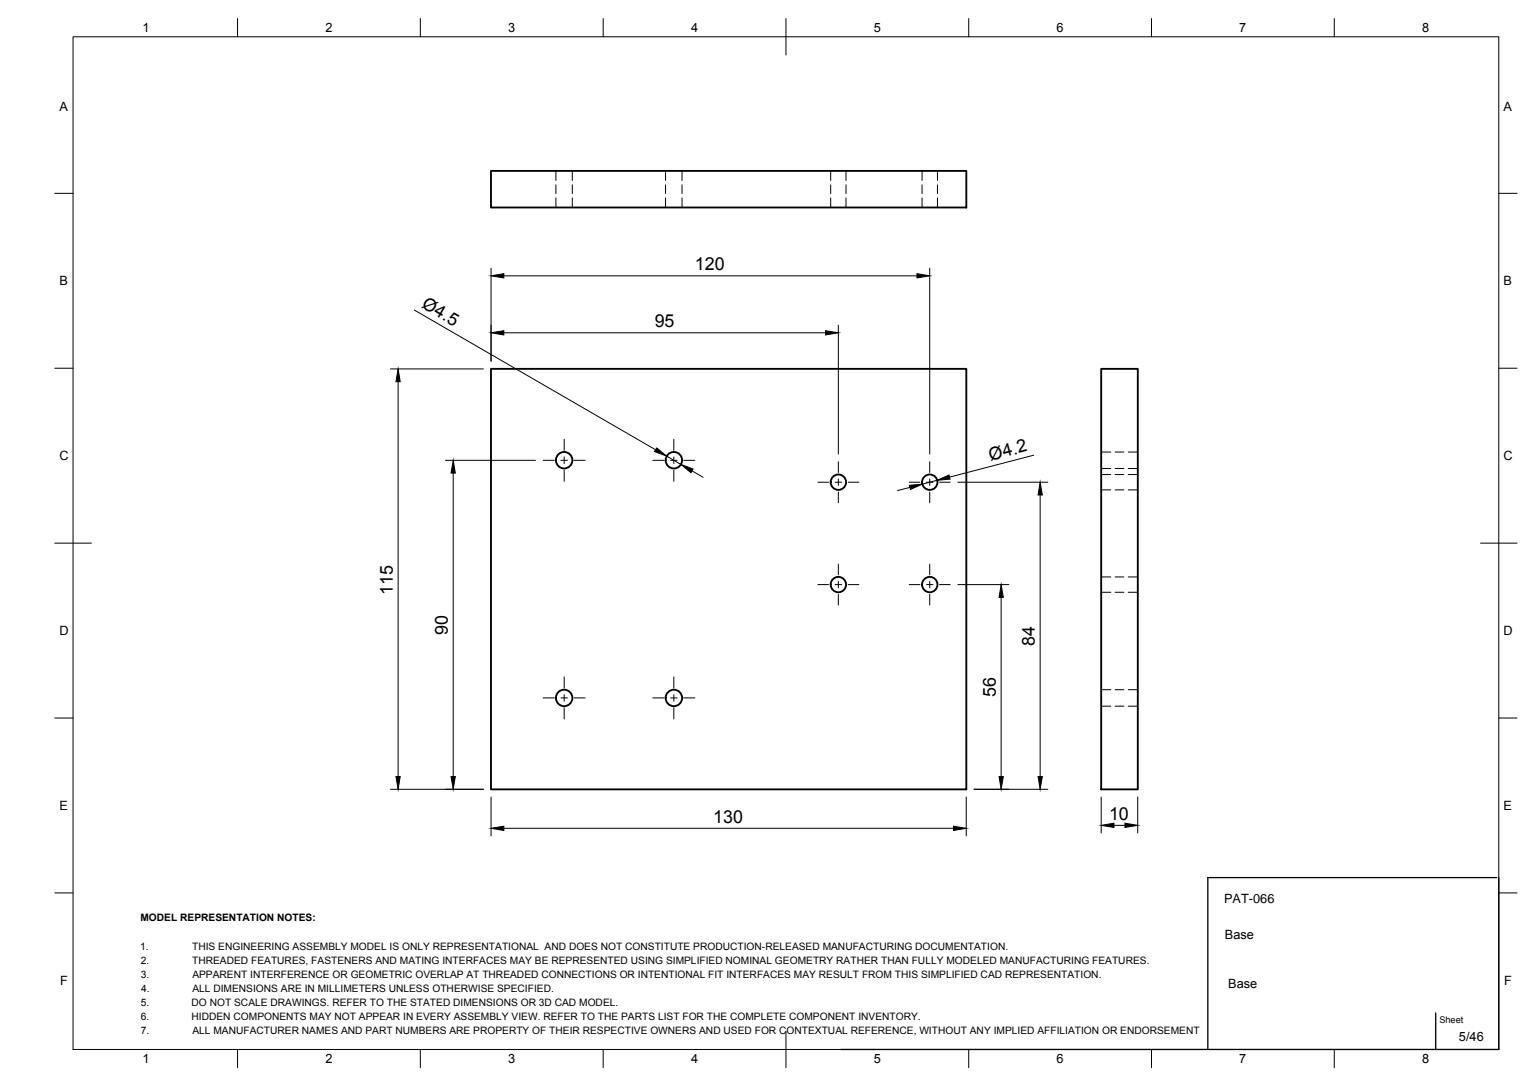
ISO-10303-21;
HEADER;
/* Generated by software containing ST-Developer
 * from STEP Tools, Inc. (www.steptools.com) 
 */

FILE_DESCRIPTION(
/* description */ ('Lever-operated bar clamp (toggle)'),
/* implementation_level */ '2;1');

FILE_NAME(
/* name */ 'Base.step',
/* time_stamp */ '2026-10-28T03:25:02-07:00',
/* author */ (''),
/* organization */ (''),
/* preprocessor_version */ 'ST-DEVELOPER v20.2',
/* originating_system */ 'Autodesk Translation Framework v15.17.0.0',
/* authorisation */ '');

FILE_SCHEMA (('AUTOMOTIVE_DESIGN { 1 0 10303 214 3 1 1 }'));
ENDSEC;

DATA;
#10=MECHANICAL_DESIGN_GEOMETRIC_PRESENTATION_REPRESENTATION('',(#410),#12413);
#334=SHAPE_REPRESENTATION_RELATIONSHIP('SRR','None',#12573,#372);
#372=ADVANCED_BREP_SHAPE_REPRESENTATION('',(#457),#12370);
#410=STYLED_ITEM('',(#12848),#457);
#457=MANIFOLD_SOLID_BREP('Body1',#6569);
#500=FACE_BOUND('',#1307,.T.);
#501=FACE_BOUND('',#1308,.T.);
#502=FACE_BOUND('',#1309,.T.);
#503=FACE_BOUND('',#1310,.T.);
#504=FACE_BOUND('',#1311,.T.);
#505=FACE_BOUND('',#1312,.T.);
#506=FACE_BOUND('',#1313,.T.);
#507=FACE_BOUND('',#1314,.T.);
#508=FACE_BOUND('',#1316,.T.);
#509=FACE_BOUND('',#1317,.T.);
#510=FACE_BOUND('',#1318,.T.);
#511=FACE_BOUND('',#1319,.T.);
#512=FACE_BOUND('',#1320,.T.);
#513=FACE_BOUND('',#1321,.T.);
#514=FACE_BOUND('',#1322,.T.);
#515=FACE_BOUND('',#1323,.T.);
#651=PLANE('',#7066);
#652=PLANE('',#7067);
#653=PLANE('',#7068);
#654=PLANE('',#7069);
#655=PLANE('',#7070);
#656=PLANE('',#7071);
#888=FACE_OUTER_BOUND('',#1294,.T.);
#889=FACE_OUTER_BOUND('',#1295,.T.);
#890=FACE_OUTER_BOUND('',#1296,.T.);
#891=FACE_OUTER_BOUND('',#1297,.T.);
#892=FACE_OUTER_BOUND('',#1298,.T.);
#893=FACE_OUTER_BOUND('',#1299,.T.);
#894=FACE_OUTER_BOUND('',#1300,.T.);
#895=FACE_OUTER_BOUND('',#1301,.T.);
#896=FACE_OUTER_BOUND('',#1302,.T.);
#897=FACE_OUTER_BOUND('',#1303,.T.);
#898=FACE_OUTER_BOUND('',#1304,.T.);
#899=FACE_OUTER_BOUND('',#1305,.T.);
#900=FACE_OUTER_BOUND('',#1306,.T.);
#901=FACE_OUTER_BOUND('',#1315,.T.);
#1294=EDGE_LOOP('',(#4421,#4422,#4423,#4424));
#1295=EDGE_LOOP('',(#4425,#4426,#4427,#4428));
#1296=EDGE_LOOP('',(#4429,#4430,#4431,#4432));
#1297=EDGE_LOOP('',(#4433,#4434,#4435,#4436));
#1298=EDGE_LOOP('',(#4437,#4438,#4439,#4440));
#1299=EDGE_LOOP('',(#4441,#4442,#4443,#4444));
#1300=EDGE_LOOP('',(#4445,#4446,#4447,#4448));
#1301=EDGE_LOOP('',(#4449,#4450,#4451,#4452));
#1302=EDGE_LOOP('',(#4453,#4454,#4455,#4456));
#1303=EDGE_LOOP('',(#4457,#4458,#4459,#4460));
#1304=EDGE_LOOP('',(#4461,#4462,#4463,#4464));
#1305=EDGE_LOOP('',(#4465,#4466,#4467,#4468));
#1306=EDGE_LOOP('',(#4469,#4470,#4471,#4472));
#1307=EDGE_LOOP('',(#4473));
#1308=EDGE_LOOP('',(#4474));
#1309=EDGE_LOOP('',(#4475));
#1310=EDGE_LOOP('',(#4476));
#1311=EDGE_LOOP('',(#4477));
#1312=EDGE_LOOP('',(#4478));
#1313=EDGE_LOOP('',(#4479));
#1314=EDGE_LOOP('',(#4480));
#1315=EDGE_LOOP('',(#4481,#4482,#4483,#4484));
#1316=EDGE_LOOP('',(#4485));
#1317=EDGE_LOOP('',(#4486));
#1318=EDGE_LOOP('',(#4487));
#1319=EDGE_LOOP('',(#4488));
#1320=EDGE_LOOP('',(#4489));
#1321=EDGE_LOOP('',(#4490));
#1322=EDGE_LOOP('',(#4491));
#1323=EDGE_LOOP('',(#4492));
#1851=LINE('',#10052,#2292);
#1852=LINE('',#10058,#2293);
#1853=LINE('',#10064,#2294);
#1854=LINE('',#10070,#2295);
#1855=LINE('',#10076,#2296);
#1856=LINE('',#10082,#2297);
#1857=LINE('',#10088,#2298);
#1858=LINE('',#10094,#2299);
#1859=LINE('',#10099,#2300);
#1860=LINE('',#10101,#2301);
#1861=LINE('',#10103,#2302);
#1862=LINE('',#10104,#2303);
#1863=LINE('',#10107,#2304);
#1864=LINE('',#10109,#2305);
#1865=LINE('',#10110,#2306);
#1866=LINE('',#10113,#2307);
#1867=LINE('',#10115,#2308);
#1868=LINE('',#10116,#2309);
#1869=LINE('',#10118,#2310);
#1870=LINE('',#10119,#2311);
#2292=VECTOR('',#7904,0.225);
#2293=VECTOR('',#7911,0.225);
#2294=VECTOR('',#7918,0.225);
#2295=VECTOR('',#7925,0.225);
#2296=VECTOR('',#7932,0.21);
#2297=VECTOR('',#7939,0.210000000000001);
#2298=VECTOR('',#7946,0.210000000000001);
#2299=VECTOR('',#7953,0.21);
#2300=VECTOR('',#7958,1.);
#2301=VECTOR('',#7959,1.);
#2302=VECTOR('',#7960,1.);
#2303=VECTOR('',#7961,1.);
#2304=VECTOR('',#7964,1.);
#2305=VECTOR('',#7965,1.);
#2306=VECTOR('',#7966,1.);
#2307=VECTOR('',#7969,1.);
#2308=VECTOR('',#7970,1.);
#2309=VECTOR('',#7971,1.);
#2310=VECTOR('',#7974,1.);
#2311=VECTOR('',#7975,1.);
#2733=CIRCLE('',#7043,0.225);
#2734=CIRCLE('',#7044,0.225);
#2735=CIRCLE('',#7046,0.225);
#2736=CIRCLE('',#7047,0.225);
#2737=CIRCLE('',#7049,0.225);
#2738=CIRCLE('',#7050,0.225);
#2739=CIRCLE('',#7052,0.225);
#2740=CIRCLE('',#7053,0.225);
#2741=CIRCLE('',#7055,0.21);
#2742=CIRCLE('',#7056,0.21);
#2743=CIRCLE('',#7058,0.210000000000001);
#2744=CIRCLE('',#7059,0.210000000000001);
#2745=CIRCLE('',#7061,0.210000000000001);
#2746=CIRCLE('',#7062,0.210000000000001);
#2747=CIRCLE('',#7064,0.21);
#2748=CIRCLE('',#7065,0.21);
#3074=VERTEX_POINT('',#10049);
#3075=VERTEX_POINT('',#10051);
#3076=VERTEX_POINT('',#10055);
#3077=VERTEX_POINT('',#10057);
#3078=VERTEX_POINT('',#10061);
#3079=VERTEX_POINT('',#10063);
#3080=VERTEX_POINT('',#10067);
#3081=VERTEX_POINT('',#10069);
#3082=VERTEX_POINT('',#10073);
#3083=VERTEX_POINT('',#10075);
#3084=VERTEX_POINT('',#10079);
#3085=VERTEX_POINT('',#10081);
#3086=VERTEX_POINT('',#10085);
#3087=VERTEX_POINT('',#10087);
#3088=VERTEX_POINT('',#10091);
#3089=VERTEX_POINT('',#10093);
#3090=VERTEX_POINT('',#10097);
#3091=VERTEX_POINT('',#10098);
#3092=VERTEX_POINT('',#10100);
#3093=VERTEX_POINT('',#10102);
#3094=VERTEX_POINT('',#10106);
#3095=VERTEX_POINT('',#10108);
#3096=VERTEX_POINT('',#10112);
#3097=VERTEX_POINT('',#10114);
#3615=EDGE_CURVE('',#3074,#3074,#2733,.T.);
#3616=EDGE_CURVE('',#3074,#3075,#1851,.T.);
#3617=EDGE_CURVE('',#3075,#3075,#2734,.T.);
#3618=EDGE_CURVE('',#3076,#3076,#2735,.T.);
#3619=EDGE_CURVE('',#3076,#3077,#1852,.T.);
#3620=EDGE_CURVE('',#3077,#3077,#2736,.T.);
#3621=EDGE_CURVE('',#3078,#3078,#2737,.T.);
#3622=EDGE_CURVE('',#3078,#3079,#1853,.T.);
#3623=EDGE_CURVE('',#3079,#3079,#2738,.T.);
#3624=EDGE_CURVE('',#3080,#3080,#2739,.T.);
#3625=EDGE_CURVE('',#3080,#3081,#1854,.T.);
#3626=EDGE_CURVE('',#3081,#3081,#2740,.T.);
#3627=EDGE_CURVE('',#3082,#3082,#2741,.T.);
#3628=EDGE_CURVE('',#3082,#3083,#1855,.T.);
#3629=EDGE_CURVE('',#3083,#3083,#2742,.T.);
#3630=EDGE_CURVE('',#3084,#3084,#2743,.T.);
#3631=EDGE_CURVE('',#3084,#3085,#1856,.T.);
#3632=EDGE_CURVE('',#3085,#3085,#2744,.T.);
#3633=EDGE_CURVE('',#3086,#3086,#2745,.T.);
#3634=EDGE_CURVE('',#3086,#3087,#1857,.T.);
#3635=EDGE_CURVE('',#3087,#3087,#2746,.T.);
#3636=EDGE_CURVE('',#3088,#3088,#2747,.T.);
#3637=EDGE_CURVE('',#3088,#3089,#1858,.T.);
#3638=EDGE_CURVE('',#3089,#3089,#2748,.T.);
#3639=EDGE_CURVE('',#3090,#3091,#1859,.T.);
#3640=EDGE_CURVE('',#3091,#3092,#1860,.T.);
#3641=EDGE_CURVE('',#3093,#3092,#1861,.T.);
#3642=EDGE_CURVE('',#3090,#3093,#1862,.T.);
#3643=EDGE_CURVE('',#3094,#3090,#1863,.T.);
#3644=EDGE_CURVE('',#3095,#3093,#1864,.T.);
#3645=EDGE_CURVE('',#3094,#3095,#1865,.T.);
#3646=EDGE_CURVE('',#3096,#3094,#1866,.T.);
#3647=EDGE_CURVE('',#3097,#3095,#1867,.T.);
#3648=EDGE_CURVE('',#3096,#3097,#1868,.T.);
#3649=EDGE_CURVE('',#3091,#3096,#1869,.T.);
#3650=EDGE_CURVE('',#3092,#3097,#1870,.T.);
#4421=ORIENTED_EDGE('',*,*,#3615,.F.);
#4422=ORIENTED_EDGE('',*,*,#3616,.T.);
#4423=ORIENTED_EDGE('',*,*,#3617,.F.);
#4424=ORIENTED_EDGE('',*,*,#3616,.F.);
#4425=ORIENTED_EDGE('',*,*,#3618,.F.);
#4426=ORIENTED_EDGE('',*,*,#3619,.T.);
#4427=ORIENTED_EDGE('',*,*,#3620,.F.);
#4428=ORIENTED_EDGE('',*,*,#3619,.F.);
#4429=ORIENTED_EDGE('',*,*,#3621,.F.);
#4430=ORIENTED_EDGE('',*,*,#3622,.T.);
#4431=ORIENTED_EDGE('',*,*,#3623,.F.);
#4432=ORIENTED_EDGE('',*,*,#3622,.F.);
#4433=ORIENTED_EDGE('',*,*,#3624,.F.);
#4434=ORIENTED_EDGE('',*,*,#3625,.T.);
#4435=ORIENTED_EDGE('',*,*,#3626,.F.);
#4436=ORIENTED_EDGE('',*,*,#3625,.F.);
#4437=ORIENTED_EDGE('',*,*,#3627,.F.);
#4438=ORIENTED_EDGE('',*,*,#3628,.T.);
#4439=ORIENTED_EDGE('',*,*,#3629,.F.);
#4440=ORIENTED_EDGE('',*,*,#3628,.F.);
#4441=ORIENTED_EDGE('',*,*,#3630,.F.);
#4442=ORIENTED_EDGE('',*,*,#3631,.T.);
#4443=ORIENTED_EDGE('',*,*,#3632,.F.);
#4444=ORIENTED_EDGE('',*,*,#3631,.F.);
#4445=ORIENTED_EDGE('',*,*,#3633,.F.);
#4446=ORIENTED_EDGE('',*,*,#3634,.T.);
#4447=ORIENTED_EDGE('',*,*,#3635,.F.);
#4448=ORIENTED_EDGE('',*,*,#3634,.F.);
#4449=ORIENTED_EDGE('',*,*,#3636,.F.);
#4450=ORIENTED_EDGE('',*,*,#3637,.T.);
#4451=ORIENTED_EDGE('',*,*,#3638,.F.);
#4452=ORIENTED_EDGE('',*,*,#3637,.F.);
#4453=ORIENTED_EDGE('',*,*,#3639,.T.);
#4454=ORIENTED_EDGE('',*,*,#3640,.T.);
#4455=ORIENTED_EDGE('',*,*,#3641,.F.);
#4456=ORIENTED_EDGE('',*,*,#3642,.F.);
#4457=ORIENTED_EDGE('',*,*,#3643,.T.);
#4458=ORIENTED_EDGE('',*,*,#3642,.T.);
#4459=ORIENTED_EDGE('',*,*,#3644,.F.);
#4460=ORIENTED_EDGE('',*,*,#3645,.F.);
#4461=ORIENTED_EDGE('',*,*,#3646,.T.);
#4462=ORIENTED_EDGE('',*,*,#3645,.T.);
#4463=ORIENTED_EDGE('',*,*,#3647,.F.);
#4464=ORIENTED_EDGE('',*,*,#3648,.F.);
#4465=ORIENTED_EDGE('',*,*,#3649,.T.);
#4466=ORIENTED_EDGE('',*,*,#3648,.T.);
#4467=ORIENTED_EDGE('',*,*,#3650,.F.);
#4468=ORIENTED_EDGE('',*,*,#3640,.F.);
#4469=ORIENTED_EDGE('',*,*,#3650,.T.);
#4470=ORIENTED_EDGE('',*,*,#3647,.T.);
#4471=ORIENTED_EDGE('',*,*,#3644,.T.);
#4472=ORIENTED_EDGE('',*,*,#3641,.T.);
#4473=ORIENTED_EDGE('',*,*,#3638,.T.);
#4474=ORIENTED_EDGE('',*,*,#3635,.T.);
#4475=ORIENTED_EDGE('',*,*,#3632,.T.);
#4476=ORIENTED_EDGE('',*,*,#3629,.T.);
#4477=ORIENTED_EDGE('',*,*,#3626,.T.);
#4478=ORIENTED_EDGE('',*,*,#3623,.T.);
#4479=ORIENTED_EDGE('',*,*,#3620,.T.);
#4480=ORIENTED_EDGE('',*,*,#3617,.T.);
#4481=ORIENTED_EDGE('',*,*,#3649,.F.);
#4482=ORIENTED_EDGE('',*,*,#3639,.F.);
#4483=ORIENTED_EDGE('',*,*,#3643,.F.);
#4484=ORIENTED_EDGE('',*,*,#3646,.F.);
#4485=ORIENTED_EDGE('',*,*,#3636,.T.);
#4486=ORIENTED_EDGE('',*,*,#3633,.T.);
#4487=ORIENTED_EDGE('',*,*,#3630,.T.);
#4488=ORIENTED_EDGE('',*,*,#3627,.T.);
#4489=ORIENTED_EDGE('',*,*,#3624,.T.);
#4490=ORIENTED_EDGE('',*,*,#3621,.T.);
#4491=ORIENTED_EDGE('',*,*,#3618,.T.);
#4492=ORIENTED_EDGE('',*,*,#3615,.T.);
#6033=CYLINDRICAL_SURFACE('',#7042,0.225);
#6034=CYLINDRICAL_SURFACE('',#7045,0.225);
#6035=CYLINDRICAL_SURFACE('',#7048,0.225);
#6036=CYLINDRICAL_SURFACE('',#7051,0.225);
#6037=CYLINDRICAL_SURFACE('',#7054,0.21);
#6038=CYLINDRICAL_SURFACE('',#7057,0.210000000000001);
#6039=CYLINDRICAL_SURFACE('',#7060,0.210000000000001);
#6040=CYLINDRICAL_SURFACE('',#7063,0.21);
#6163=ADVANCED_FACE('',(#888),#6033,.F.);
#6164=ADVANCED_FACE('',(#889),#6034,.F.);
#6165=ADVANCED_FACE('',(#890),#6035,.F.);
#6166=ADVANCED_FACE('',(#891),#6036,.F.);
#6167=ADVANCED_FACE('',(#892),#6037,.F.);
#6168=ADVANCED_FACE('',(#893),#6038,.F.);
#6169=ADVANCED_FACE('',(#894),#6039,.F.);
#6170=ADVANCED_FACE('',(#895),#6040,.F.);
#6171=ADVANCED_FACE('',(#896),#651,.T.);
#6172=ADVANCED_FACE('',(#897),#652,.T.);
#6173=ADVANCED_FACE('',(#898),#653,.T.);
#6174=ADVANCED_FACE('',(#899),#654,.T.);
#6175=ADVANCED_FACE('',(#900,#500,#501,#502,#503,#504,#505,#506,#507),#655,
 .T.);
#6176=ADVANCED_FACE('',(#901,#508,#509,#510,#511,#512,#513,#514,#515),#656,
 .F.);
#6569=CLOSED_SHELL('',(#6163,#6164,#6165,#6166,#6167,#6168,#6169,#6170,
#6171,#6172,#6173,#6174,#6175,#6176));
#7041=AXIS2_PLACEMENT_3D('',#10047,#7898,#7899);
#7042=AXIS2_PLACEMENT_3D('',#10048,#7900,#7901);
#7043=AXIS2_PLACEMENT_3D('',#10050,#7902,#7903);
#7044=AXIS2_PLACEMENT_3D('',#10053,#7905,#7906);
#7045=AXIS2_PLACEMENT_3D('',#10054,#7907,#7908);
#7046=AXIS2_PLACEMENT_3D('',#10056,#7909,#7910);
#7047=AXIS2_PLACEMENT_3D('',#10059,#7912,#7913);
#7048=AXIS2_PLACEMENT_3D('',#10060,#7914,#7915);
#7049=AXIS2_PLACEMENT_3D('',#10062,#7916,#7917);
#7050=AXIS2_PLACEMENT_3D('',#10065,#7919,#7920);
#7051=AXIS2_PLACEMENT_3D('',#10066,#7921,#7922);
#7052=AXIS2_PLACEMENT_3D('',#10068,#7923,#7924);
#7053=AXIS2_PLACEMENT_3D('',#10071,#7926,#7927);
#7054=AXIS2_PLACEMENT_3D('',#10072,#7928,#7929);
#7055=AXIS2_PLACEMENT_3D('',#10074,#7930,#7931);
#7056=AXIS2_PLACEMENT_3D('',#10077,#7933,#7934);
#7057=AXIS2_PLACEMENT_3D('',#10078,#7935,#7936);
#7058=AXIS2_PLACEMENT_3D('',#10080,#7937,#7938);
#7059=AXIS2_PLACEMENT_3D('',#10083,#7940,#7941);
#7060=AXIS2_PLACEMENT_3D('',#10084,#7942,#7943);
#7061=AXIS2_PLACEMENT_3D('',#10086,#7944,#7945);
#7062=AXIS2_PLACEMENT_3D('',#10089,#7947,#7948);
#7063=AXIS2_PLACEMENT_3D('',#10090,#7949,#7950);
#7064=AXIS2_PLACEMENT_3D('',#10092,#7951,#7952);
#7065=AXIS2_PLACEMENT_3D('',#10095,#7954,#7955);
#7066=AXIS2_PLACEMENT_3D('',#10096,#7956,#7957);
#7067=AXIS2_PLACEMENT_3D('',#10105,#7962,#7963);
#7068=AXIS2_PLACEMENT_3D('',#10111,#7967,#7968);
#7069=AXIS2_PLACEMENT_3D('',#10117,#7972,#7973);
#7070=AXIS2_PLACEMENT_3D('',#10120,#7976,#7977);
#7071=AXIS2_PLACEMENT_3D('',#10121,#7978,#7979);
#7898=DIRECTION('axis',(0.,0.,1.));
#7899=DIRECTION('refdir',(1.,0.,0.));
#7900=DIRECTION('center_axis',(0.,0.,1.));
#7901=DIRECTION('ref_axis',(1.,0.,0.));
#7902=DIRECTION('center_axis',(0.,0.,1.));
#7903=DIRECTION('ref_axis',(1.,0.,0.));
#7904=DIRECTION('',(0.,0.,1.));
#7905=DIRECTION('center_axis',(0.,0.,-1.));
#7906=DIRECTION('ref_axis',(1.,0.,0.));
#7907=DIRECTION('center_axis',(0.,0.,1.));
#7908=DIRECTION('ref_axis',(1.,0.,0.));
#7909=DIRECTION('center_axis',(0.,0.,1.));
#7910=DIRECTION('ref_axis',(1.,0.,0.));
#7911=DIRECTION('',(0.,0.,1.));
#7912=DIRECTION('center_axis',(0.,0.,-1.));
#7913=DIRECTION('ref_axis',(1.,0.,0.));
#7914=DIRECTION('center_axis',(0.,0.,1.));
#7915=DIRECTION('ref_axis',(1.,0.,0.));
#7916=DIRECTION('center_axis',(0.,0.,1.));
#7917=DIRECTION('ref_axis',(1.,0.,0.));
#7918=DIRECTION('',(0.,0.,1.));
#7919=DIRECTION('center_axis',(0.,0.,-1.));
#7920=DIRECTION('ref_axis',(1.,0.,0.));
#7921=DIRECTION('center_axis',(0.,0.,1.));
#7922=DIRECTION('ref_axis',(1.,0.,0.));
#7923=DIRECTION('center_axis',(0.,0.,1.));
#7924=DIRECTION('ref_axis',(1.,0.,0.));
#7925=DIRECTION('',(0.,0.,1.));
#7926=DIRECTION('center_axis',(0.,0.,-1.));
#7927=DIRECTION('ref_axis',(1.,0.,0.));
#7928=DIRECTION('center_axis',(0.,0.,1.));
#7929=DIRECTION('ref_axis',(1.,0.,0.));
#7930=DIRECTION('center_axis',(0.,0.,1.));
#7931=DIRECTION('ref_axis',(1.,0.,0.));
#7932=DIRECTION('',(0.,0.,1.));
#7933=DIRECTION('center_axis',(0.,0.,-1.));
#7934=DIRECTION('ref_axis',(1.,0.,0.));
#7935=DIRECTION('center_axis',(0.,0.,1.));
#7936=DIRECTION('ref_axis',(1.,0.,0.));
#7937=DIRECTION('center_axis',(0.,0.,1.));
#7938=DIRECTION('ref_axis',(1.,0.,0.));
#7939=DIRECTION('',(0.,0.,1.));
#7940=DIRECTION('center_axis',(0.,0.,-1.));
#7941=DIRECTION('ref_axis',(1.,0.,0.));
#7942=DIRECTION('center_axis',(0.,0.,1.));
#7943=DIRECTION('ref_axis',(1.,0.,0.));
#7944=DIRECTION('center_axis',(0.,0.,1.));
#7945=DIRECTION('ref_axis',(1.,0.,0.));
#7946=DIRECTION('',(0.,0.,1.));
#7947=DIRECTION('center_axis',(0.,0.,-1.));
#7948=DIRECTION('ref_axis',(1.,0.,0.));
#7949=DIRECTION('center_axis',(0.,0.,1.));
#7950=DIRECTION('ref_axis',(1.,0.,0.));
#7951=DIRECTION('center_axis',(0.,0.,1.));
#7952=DIRECTION('ref_axis',(1.,0.,0.));
#7953=DIRECTION('',(0.,0.,1.));
#7954=DIRECTION('center_axis',(0.,0.,-1.));
#7955=DIRECTION('ref_axis',(1.,0.,0.));
#7956=DIRECTION('center_axis',(0.,1.,0.));
#7957=DIRECTION('ref_axis',(-1.,0.,0.));
#7958=DIRECTION('',(-1.,0.,0.));
#7959=DIRECTION('',(0.,0.,1.));
#7960=DIRECTION('',(-1.,0.,0.));
#7961=DIRECTION('',(0.,0.,1.));
#7962=DIRECTION('center_axis',(1.,0.,0.));
#7963=DIRECTION('ref_axis',(0.,1.,0.));
#7964=DIRECTION('',(0.,1.,0.));
#7965=DIRECTION('',(0.,1.,0.));
#7966=DIRECTION('',(0.,0.,1.));
#7967=DIRECTION('center_axis',(0.,-1.,0.));
#7968=DIRECTION('ref_axis',(1.,0.,0.));
#7969=DIRECTION('',(1.,0.,0.));
#7970=DIRECTION('',(1.,0.,0.));
#7971=DIRECTION('',(0.,0.,1.));
#7972=DIRECTION('center_axis',(-1.,0.,0.));
#7973=DIRECTION('ref_axis',(0.,-1.,0.));
#7974=DIRECTION('',(0.,-1.,0.));
#7975=DIRECTION('',(0.,-1.,0.));
#7976=DIRECTION('center_axis',(0.,0.,1.));
#7977=DIRECTION('ref_axis',(1.,0.,0.));
#7978=DIRECTION('center_axis',(0.,0.,1.));
#7979=DIRECTION('ref_axis',(1.,0.,0.));
#10047=CARTESIAN_POINT('',(0.,0.,0.));
#10048=CARTESIAN_POINT('Origin',(1.5,-4.5,-0.1));
#10049=CARTESIAN_POINT('',(1.275,-4.5,0.));
#10050=CARTESIAN_POINT('Origin',(1.5,-4.5,0.));
#10051=CARTESIAN_POINT('',(1.275,-4.5,1.));
#10052=CARTESIAN_POINT('',(1.275,-4.5,-0.1));
#10053=CARTESIAN_POINT('Origin',(1.5,-4.5,1.));
#10054=CARTESIAN_POINT('Origin',(1.5,2.,-0.1));
#10055=CARTESIAN_POINT('',(1.275,2.,0.));
#10056=CARTESIAN_POINT('Origin',(1.5,2.,0.));
#10057=CARTESIAN_POINT('',(1.275,2.,1.));
#10058=CARTESIAN_POINT('',(1.275,2.,-0.1));
#10059=CARTESIAN_POINT('Origin',(1.5,2.,1.));
#10060=CARTESIAN_POINT('Origin',(-1.5,-4.5,-0.1));
#10061=CARTESIAN_POINT('',(-1.725,-4.5,0.));
#10062=CARTESIAN_POINT('Origin',(-1.5,-4.5,0.));
#10063=CARTESIAN_POINT('',(-1.725,-4.5,1.));
#10064=CARTESIAN_POINT('',(-1.725,-4.5,-0.1));
#10065=CARTESIAN_POINT('Origin',(-1.5,-4.5,1.));
#10066=CARTESIAN_POINT('Origin',(-1.5,2.,-0.1));
#10067=CARTESIAN_POINT('',(-1.725,2.,0.));
#10068=CARTESIAN_POINT('Origin',(-1.5,2.,0.));
#10069=CARTESIAN_POINT('',(-1.725,2.,1.));
#10070=CARTESIAN_POINT('',(-1.725,2.,-0.1));
#10071=CARTESIAN_POINT('Origin',(-1.5,2.,1.));
#10072=CARTESIAN_POINT('Origin',(-6.,-1.4,-0.1));
#10073=CARTESIAN_POINT('',(-6.21,-1.4,0.));
#10074=CARTESIAN_POINT('Origin',(-6.,-1.4,0.));
#10075=CARTESIAN_POINT('',(-6.21,-1.4,1.));
#10076=CARTESIAN_POINT('',(-6.21,-1.4,-0.1));
#10077=CARTESIAN_POINT('Origin',(-6.,-1.4,1.));
#10078=CARTESIAN_POINT('Origin',(-8.5,1.4,-0.1));
#10079=CARTESIAN_POINT('',(-8.71,1.4,0.));
#10080=CARTESIAN_POINT('Origin',(-8.5,1.4,0.));
#10081=CARTESIAN_POINT('',(-8.71,1.4,1.));
#10082=CARTESIAN_POINT('',(-8.71,1.4,-0.1));
#10083=CARTESIAN_POINT('Origin',(-8.5,1.4,1.));
#10084=CARTESIAN_POINT('Origin',(-8.5,-1.4,-0.1));
#10085=CARTESIAN_POINT('',(-8.71,-1.4,0.));
#10086=CARTESIAN_POINT('Origin',(-8.5,-1.4,0.));
#10087=CARTESIAN_POINT('',(-8.71,-1.4,1.));
#10088=CARTESIAN_POINT('',(-8.71,-1.4,-0.1));
#10089=CARTESIAN_POINT('Origin',(-8.5,-1.4,1.));
#10090=CARTESIAN_POINT('Origin',(-6.,1.4,-0.1));
#10091=CARTESIAN_POINT('',(-6.21,1.4,0.));
#10092=CARTESIAN_POINT('Origin',(-6.,1.4,0.));
#10093=CARTESIAN_POINT('',(-6.21,1.4,1.));
#10094=CARTESIAN_POINT('',(-6.21,1.4,-0.1));
#10095=CARTESIAN_POINT('Origin',(-6.,1.4,1.));
#10096=CARTESIAN_POINT('Origin',(3.5,4.5,0.));
#10097=CARTESIAN_POINT('',(3.5,4.5,0.));
#10098=CARTESIAN_POINT('',(-9.5,4.5,0.));
#10099=CARTESIAN_POINT('',(3.5,4.5,0.));
#10100=CARTESIAN_POINT('',(-9.5,4.5,1.));
#10101=CARTESIAN_POINT('',(-9.5,4.5,0.));
#10102=CARTESIAN_POINT('',(3.5,4.5,1.));
#10103=CARTESIAN_POINT('',(3.5,4.5,1.));
#10104=CARTESIAN_POINT('',(3.5,4.5,0.));
#10105=CARTESIAN_POINT('Origin',(3.5,-7.,0.));
#10106=CARTESIAN_POINT('',(3.5,-7.,0.));
#10107=CARTESIAN_POINT('',(3.5,-7.,0.));
#10108=CARTESIAN_POINT('',(3.5,-7.,1.));
#10109=CARTESIAN_POINT('',(3.5,-7.,1.));
#10110=CARTESIAN_POINT('',(3.5,-7.,0.));
#10111=CARTESIAN_POINT('Origin',(-9.5,-7.,0.));
#10112=CARTESIAN_POINT('',(-9.5,-7.,0.));
#10113=CARTESIAN_POINT('',(-9.5,-7.,0.));
#10114=CARTESIAN_POINT('',(-9.5,-7.,1.));
#10115=CARTESIAN_POINT('',(-9.5,-7.,1.));
#10116=CARTESIAN_POINT('',(-9.5,-7.,0.));
#10117=CARTESIAN_POINT('Origin',(-9.5,4.5,0.));
#10118=CARTESIAN_POINT('',(-9.5,4.5,0.));
#10119=CARTESIAN_POINT('',(-9.5,4.5,1.));
#10120=CARTESIAN_POINT('Origin',(-3.,-1.25,1.));
#10121=CARTESIAN_POINT('Origin',(-3.,-1.25,0.));
#12324=UNCERTAINTY_MEASURE_WITH_UNIT(LENGTH_MEASURE(0.001),#12414,
'DISTANCE_ACCURACY_VALUE',
'Maximum model space distance between geometric entities at asserted c
onnectivities');
#12367=UNCERTAINTY_MEASURE_WITH_UNIT(LENGTH_MEASURE(0.001),#12414,
'DISTANCE_ACCURACY_VALUE',
'Maximum model space distance between geometric entities at asserted c
onnectivities');
#12370=(
GEOMETRIC_REPRESENTATION_CONTEXT(3)
GLOBAL_UNCERTAINTY_ASSIGNED_CONTEXT((#12324))
GLOBAL_UNIT_ASSIGNED_CONTEXT((#12414,#12416,#12417))
REPRESENTATION_CONTEXT('','3D')
);
#12413=(
GEOMETRIC_REPRESENTATION_CONTEXT(3)
GLOBAL_UNCERTAINTY_ASSIGNED_CONTEXT((#12367))
GLOBAL_UNIT_ASSIGNED_CONTEXT((#12414,#12416,#12417))
REPRESENTATION_CONTEXT('','3D')
);
#12414=(
LENGTH_UNIT()
NAMED_UNIT(*)
SI_UNIT(.CENTI.,.METRE.)
);
#12416=(
NAMED_UNIT(*)
PLANE_ANGLE_UNIT()
SI_UNIT($,.RADIAN.)
);
#12417=(
NAMED_UNIT(*)
SI_UNIT($,.STERADIAN.)
SOLID_ANGLE_UNIT()
);
#12420=SHAPE_DEFINITION_REPRESENTATION(#12465,#12573);
#12465=PRODUCT_DEFINITION_SHAPE('',$,#12619);
#12573=SHAPE_REPRESENTATION('',(#7041),#12370);
#12616=PRODUCT_DEFINITION_CONTEXT('part definition',#12753,'design');
#12619=PRODUCT_DEFINITION('Base','Base',#12664,#12616);
#12664=PRODUCT_DEFINITION_FORMATION('',$,#12757);
#12753=APPLICATION_CONTEXT(
'Core Data for Automotive Mechanical Design Process');
#12754=PRODUCT_CONTEXT('part definition',#12753,'mechanical');
#12757=PRODUCT('Base','Base','Base',(#12754));
#12842=COLOUR_RGB('Dark Blue',0.08,0.2,0.34);
#12843=FILL_AREA_STYLE_COLOUR('',#12842);
#12844=FILL_AREA_STYLE('',(#12843));
#12845=SURFACE_STYLE_FILL_AREA(#12844);
#12846=SURFACE_SIDE_STYLE('',(#12845));
#12847=SURFACE_STYLE_USAGE(.BOTH.,#12846);
#12848=PRESENTATION_STYLE_ASSIGNMENT((#12847));
ENDSEC;
END-ISO-10303-21;
